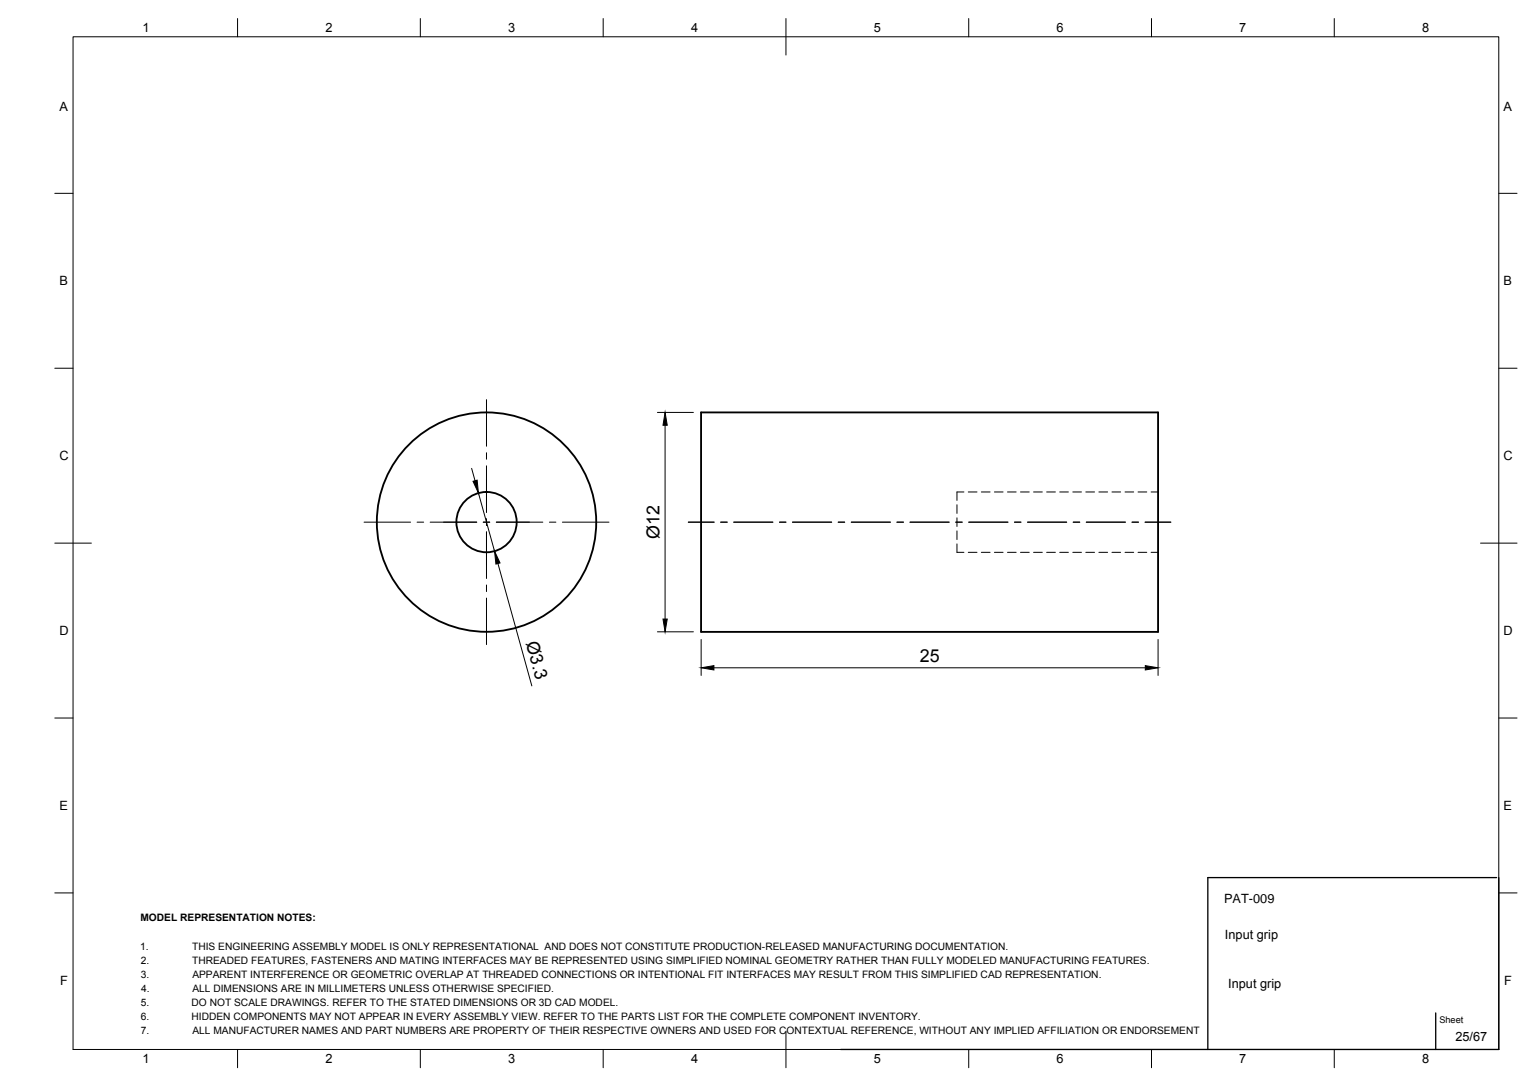
ISO-10303-21;
HEADER;
/* Generated by software containing ST-Developer
 * from STEP Tools, Inc. (www.steptools.com) 
 */

FILE_DESCRIPTION(
/* description */ ('Bell-crank linkage with push rods'),
/* implementation_level */ '2;1');

FILE_NAME(
/* name */ 'Input grip.step',
/* time_stamp */ '2026-10-28T03:25:15-07:00',
/* author */ (''),
/* organization */ (''),
/* preprocessor_version */ 'ST-DEVELOPER v20.2',
/* originating_system */ 'Autodesk Translation Framework v15.17.0.0',
/* authorisation */ '');

FILE_SCHEMA (('AUTOMOTIVE_DESIGN { 1 0 10303 214 3 1 1 }'));
ENDSEC;

DATA;
#10=MECHANICAL_DESIGN_GEOMETRIC_PRESENTATION_REPRESENTATION('',(#630),#16678);
#514=SHAPE_REPRESENTATION_RELATIONSHIP('SRR','None',#16932,#568);
#568=ADVANCED_BREP_SHAPE_REPRESENTATION('',(#691),#16637);
#630=STYLED_ITEM('',(#17298),#691);
#691=MANIFOLD_SOLID_BREP('Body1',#8821);
#831=FACE_BOUND('',#2131,.T.);
#1092=PLANE('',#9996);
#1093=PLANE('',#10000);
#1094=PLANE('',#10001);
#1498=FACE_OUTER_BOUND('',#2126,.T.);
#1499=FACE_OUTER_BOUND('',#2127,.T.);
#1500=FACE_OUTER_BOUND('',#2128,.T.);
#1501=FACE_OUTER_BOUND('',#2129,.T.);
#1502=FACE_OUTER_BOUND('',#2130,.T.);
#2126=EDGE_LOOP('',(#7049,#7050,#7051,#7052));
#2127=EDGE_LOOP('',(#7053));
#2128=EDGE_LOOP('',(#7054,#7055,#7056,#7057));
#2129=EDGE_LOOP('',(#7058));
#2130=EDGE_LOOP('',(#7059));
#2131=EDGE_LOOP('',(#7060));
#2807=LINE('',#15241,#3356);
#2808=LINE('',#15248,#3357);
#3356=VECTOR('',#11987,0.165);
#3357=VECTOR('',#11996,0.6);
#3890=CIRCLE('',#9994,0.165);
#3891=CIRCLE('',#9995,0.165);
#3892=CIRCLE('',#9998,0.6);
#3893=CIRCLE('',#9999,0.6);
#4496=VERTEX_POINT('',#15238);
#4497=VERTEX_POINT('',#15240);
#4498=VERTEX_POINT('',#15245);
#4499=VERTEX_POINT('',#15247);
#5402=EDGE_CURVE('',#4496,#4496,#3890,.T.);
#5403=EDGE_CURVE('',#4496,#4497,#2807,.T.);
#5404=EDGE_CURVE('',#4497,#4497,#3891,.T.);
#5405=EDGE_CURVE('',#4498,#4498,#3892,.T.);
#5406=EDGE_CURVE('',#4498,#4499,#2808,.T.);
#5407=EDGE_CURVE('',#4499,#4499,#3893,.T.);
#7049=ORIENTED_EDGE('',*,*,#5402,.F.);
#7050=ORIENTED_EDGE('',*,*,#5403,.T.);
#7051=ORIENTED_EDGE('',*,*,#5404,.T.);
#7052=ORIENTED_EDGE('',*,*,#5403,.F.);
#7053=ORIENTED_EDGE('',*,*,#5404,.F.);
#7054=ORIENTED_EDGE('',*,*,#5405,.F.);
#7055=ORIENTED_EDGE('',*,*,#5406,.T.);
#7056=ORIENTED_EDGE('',*,*,#5407,.T.);
#7057=ORIENTED_EDGE('',*,*,#5406,.F.);
#7058=ORIENTED_EDGE('',*,*,#5405,.T.);
#7059=ORIENTED_EDGE('',*,*,#5407,.F.);
#7060=ORIENTED_EDGE('',*,*,#5402,.T.);
#8164=CYLINDRICAL_SURFACE('',#9993,0.165);
#8165=CYLINDRICAL_SURFACE('',#9997,0.6);
#8523=ADVANCED_FACE('',(#1498),#8164,.F.);
#8524=ADVANCED_FACE('',(#1499),#1092,.F.);
#8525=ADVANCED_FACE('',(#1500),#8165,.T.);
#8526=ADVANCED_FACE('',(#1501),#1093,.T.);
#8527=ADVANCED_FACE('',(#1502,#831),#1094,.F.);
#8821=CLOSED_SHELL('',(#8523,#8524,#8525,#8526,#8527));
#9992=AXIS2_PLACEMENT_3D('',#15236,#11981,#11982);
#9993=AXIS2_PLACEMENT_3D('',#15237,#11983,#11984);
#9994=AXIS2_PLACEMENT_3D('',#15239,#11985,#11986);
#9995=AXIS2_PLACEMENT_3D('',#15242,#11988,#11989);
#9996=AXIS2_PLACEMENT_3D('',#15243,#11990,#11991);
#9997=AXIS2_PLACEMENT_3D('',#15244,#11992,#11993);
#9998=AXIS2_PLACEMENT_3D('',#15246,#11994,#11995);
#9999=AXIS2_PLACEMENT_3D('',#15249,#11997,#11998);
#10000=AXIS2_PLACEMENT_3D('',#15250,#11999,#12000);
#10001=AXIS2_PLACEMENT_3D('',#15251,#12001,#12002);
#11981=DIRECTION('axis',(0.,0.,1.));
#11982=DIRECTION('refdir',(1.,0.,0.));
#11983=DIRECTION('center_axis',(0.,0.,1.));
#11984=DIRECTION('ref_axis',(1.,0.,0.));
#11985=DIRECTION('center_axis',(0.,0.,1.));
#11986=DIRECTION('ref_axis',(1.,0.,0.));
#11987=DIRECTION('',(0.,0.,1.));
#11988=DIRECTION('center_axis',(0.,0.,1.));
#11989=DIRECTION('ref_axis',(1.,0.,0.));
#11990=DIRECTION('center_axis',(0.,0.,1.));
#11991=DIRECTION('ref_axis',(1.,0.,0.));
#11992=DIRECTION('center_axis',(0.,0.,1.));
#11993=DIRECTION('ref_axis',(1.,0.,0.));
#11994=DIRECTION('center_axis',(0.,0.,1.));
#11995=DIRECTION('ref_axis',(1.,0.,0.));
#11996=DIRECTION('',(0.,0.,-1.));
#11997=DIRECTION('center_axis',(0.,0.,1.));
#11998=DIRECTION('ref_axis',(1.,0.,0.));
#11999=DIRECTION('center_axis',(0.,0.,1.));
#12000=DIRECTION('ref_axis',(1.,0.,0.));
#12001=DIRECTION('center_axis',(0.,0.,1.));
#12002=DIRECTION('ref_axis',(1.,0.,0.));
#15236=CARTESIAN_POINT('',(0.,0.,0.));
#15237=CARTESIAN_POINT('Origin',(-2.5,-2.5,5.5));
#15238=CARTESIAN_POINT('',(-2.665,-2.5,5.6));
#15239=CARTESIAN_POINT('Origin',(-2.5,-2.5,5.6));
#15240=CARTESIAN_POINT('',(-2.665,-2.5,6.7));
#15241=CARTESIAN_POINT('',(-2.665,-2.5,5.5));
#15242=CARTESIAN_POINT('Origin',(-2.5,-2.5,6.7));
#15243=CARTESIAN_POINT('Origin',(-2.5,-2.5,6.7));
#15244=CARTESIAN_POINT('Origin',(-2.5,-2.5,5.6));
#15245=CARTESIAN_POINT('',(-3.1,-2.5,8.1));
#15246=CARTESIAN_POINT('Origin',(-2.5,-2.5,8.1));
#15247=CARTESIAN_POINT('',(-3.1,-2.5,5.6));
#15248=CARTESIAN_POINT('',(-3.1,-2.5,5.6));
#15249=CARTESIAN_POINT('Origin',(-2.5,-2.5,5.6));
#15250=CARTESIAN_POINT('Origin',(-2.5,-2.5,8.1));
#15251=CARTESIAN_POINT('Origin',(-2.5,-2.5,5.6));
#16573=UNCERTAINTY_MEASURE_WITH_UNIT(LENGTH_MEASURE(0.001),#16679,
'DISTANCE_ACCURACY_VALUE',
'Maximum model space distance between geometric entities at asserted c
onnectivities');
#16614=UNCERTAINTY_MEASURE_WITH_UNIT(LENGTH_MEASURE(0.001),#16679,
'DISTANCE_ACCURACY_VALUE',
'Maximum model space distance between geometric entities at asserted c
onnectivities');
#16637=(
GEOMETRIC_REPRESENTATION_CONTEXT(3)
GLOBAL_UNCERTAINTY_ASSIGNED_CONTEXT((#16573))
GLOBAL_UNIT_ASSIGNED_CONTEXT((#16679,#16681,#16682))
REPRESENTATION_CONTEXT('','3D')
);
#16678=(
GEOMETRIC_REPRESENTATION_CONTEXT(3)
GLOBAL_UNCERTAINTY_ASSIGNED_CONTEXT((#16614))
GLOBAL_UNIT_ASSIGNED_CONTEXT((#16679,#16681,#16682))
REPRESENTATION_CONTEXT('','3D')
);
#16679=(
LENGTH_UNIT()
NAMED_UNIT(*)
SI_UNIT(.CENTI.,.METRE.)
);
#16681=(
NAMED_UNIT(*)
PLANE_ANGLE_UNIT()
SI_UNIT($,.RADIAN.)
);
#16682=(
NAMED_UNIT(*)
SI_UNIT($,.STERADIAN.)
SOLID_ANGLE_UNIT()
);
#16705=SHAPE_DEFINITION_REPRESENTATION(#16773,#16932);
#16773=PRODUCT_DEFINITION_SHAPE('',$,#16996);
#16932=SHAPE_REPRESENTATION('',(#9992),#16637);
#16973=PRODUCT_DEFINITION_CONTEXT('part definition',#17164,'design');
#16996=PRODUCT_DEFINITION('Input grip','Input grip',#17059,#16973);
#17059=PRODUCT_DEFINITION_FORMATION('',$,#17188);
#17164=APPLICATION_CONTEXT(
'Core Data for Automotive Mechanical Design Process');
#17165=PRODUCT_CONTEXT('part definition',#17164,'mechanical');
#17188=PRODUCT('Input grip','Input grip','Input grip',(#17165));
#17292=COLOUR_RGB('Black',0.12,0.14,0.17);
#17293=FILL_AREA_STYLE_COLOUR('',#17292);
#17294=FILL_AREA_STYLE('',(#17293));
#17295=SURFACE_STYLE_FILL_AREA(#17294);
#17296=SURFACE_SIDE_STYLE('',(#17295));
#17297=SURFACE_STYLE_USAGE(.BOTH.,#17296);
#17298=PRESENTATION_STYLE_ASSIGNMENT((#17297));
ENDSEC;
END-ISO-10303-21;
